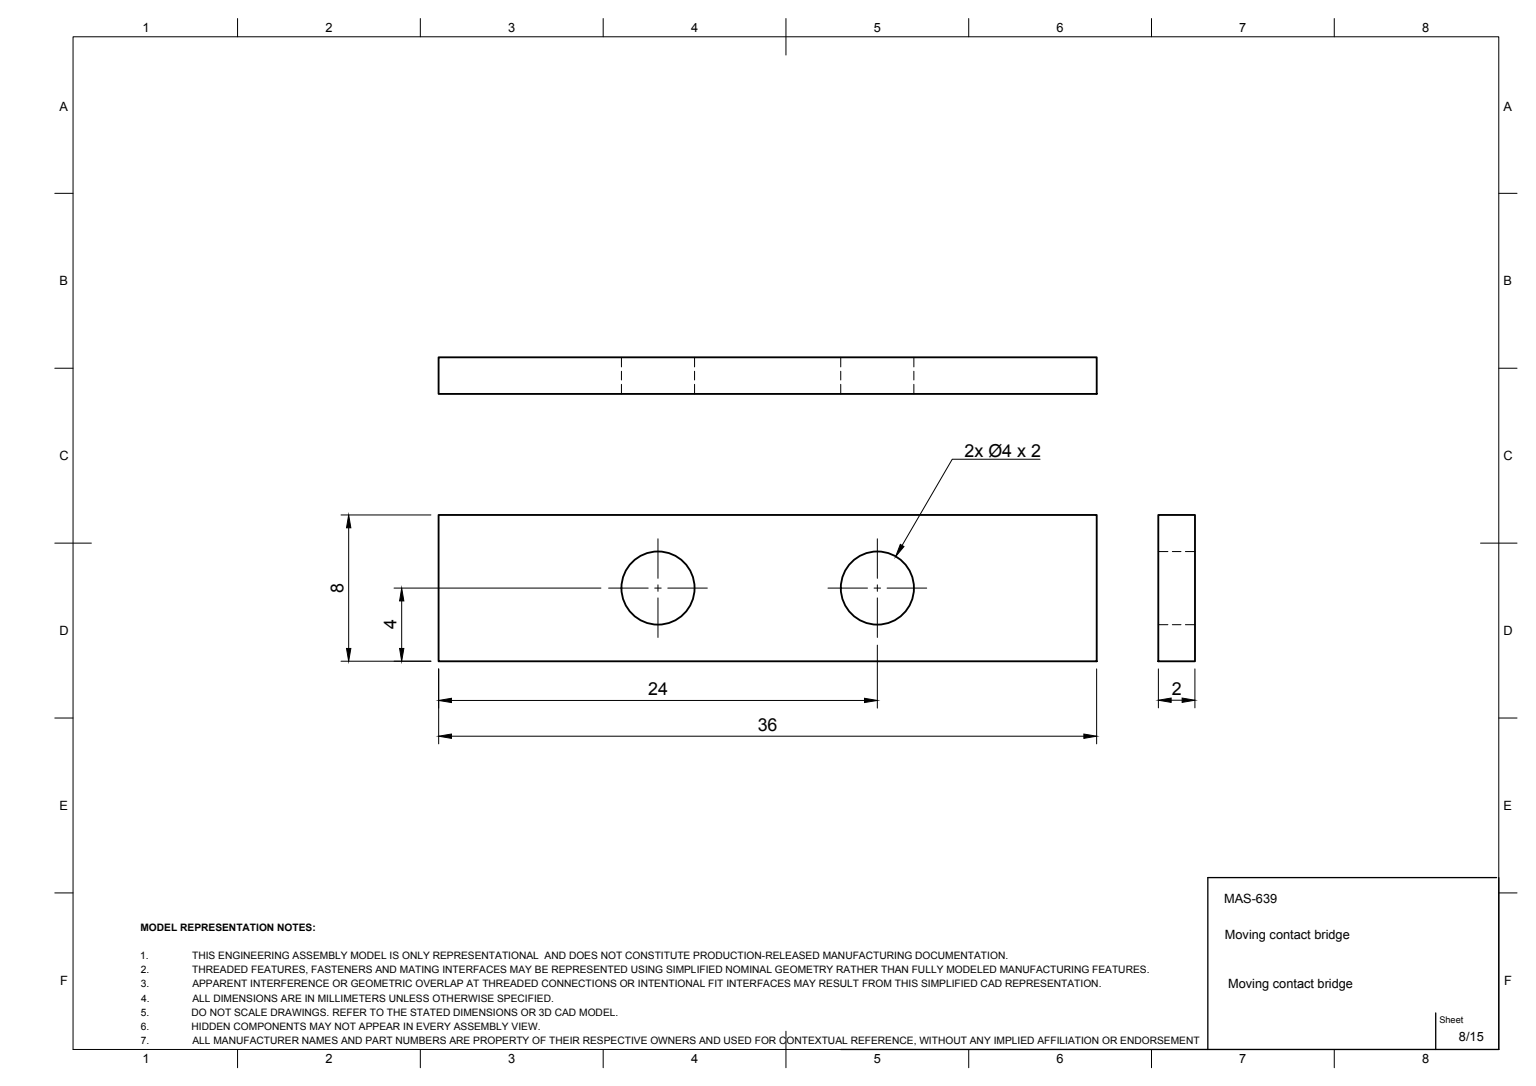
ISO-10303-21;
HEADER;
/* Generated by software containing ST-Developer
 * from STEP Tools, Inc. (www.steptools.com) 
 */

FILE_DESCRIPTION(
/* description */ ('Independent maintained push-to-latch/pull-to-reset mushroom-operator 
CAD. Two opposed spring-loaded ball detents in turned circular seats b
ias both travel stops; direct normally-closed bridge opens6mm when pre
ssed. Rounded palm/pull rim, captured head screw, removable detent clo
sures, native Coil spring families, insulated shared terminals and ord
inary machining features. Manual geometric states and ideal same-mater
ial spring-energy direction only; no electrical/safety certification, 
force/contact dynamics, wear, load or life rating. Requested blue/gray
 visual palette, not safety identification. External wiring/anchors an
d application engineering omitted.'),
/* implementation_level */ '2;1');

FILE_NAME(
/* name */ 'Moving contact bridge.step',
/* time_stamp */ '2026-11-08T17:54:26-08:00',
/* author */ (''),
/* organization */ (''),
/* preprocessor_version */ 'ST-DEVELOPER v20.2',
/* originating_system */ 'Autodesk Translation Framework v15.17.0.0',
/* authorisation */ '');

FILE_SCHEMA (('AUTOMOTIVE_DESIGN { 1 0 10303 214 3 1 1 }'));
ENDSEC;

DATA;
#10=MECHANICAL_DESIGN_GEOMETRIC_PRESENTATION_REPRESENTATION('',(#195),#43980);
#161=SHAPE_REPRESENTATION_RELATIONSHIP('SRR','None',#44061,#178);
#178=ADVANCED_BREP_SHAPE_REPRESENTATION('',(#212),#43968);
#195=STYLED_ITEM('',(#44154),#212);
#212=MANIFOLD_SOLID_BREP('Body1',#11236);
#311=FACE_BOUND('',#1491,.T.);
#312=FACE_BOUND('',#1492,.T.);
#313=FACE_BOUND('',#1494,.T.);
#314=FACE_BOUND('',#1495,.T.);
#405=PLANE('',#11885);
#406=PLANE('',#11886);
#407=PLANE('',#11887);
#408=PLANE('',#11888);
#409=PLANE('',#11889);
#410=PLANE('',#11890);
#809=FACE_OUTER_BOUND('',#1484,.T.);
#810=FACE_OUTER_BOUND('',#1485,.T.);
#811=FACE_OUTER_BOUND('',#1486,.T.);
#812=FACE_OUTER_BOUND('',#1487,.T.);
#813=FACE_OUTER_BOUND('',#1488,.T.);
#814=FACE_OUTER_BOUND('',#1489,.T.);
#815=FACE_OUTER_BOUND('',#1490,.T.);
#816=FACE_OUTER_BOUND('',#1493,.T.);
#1484=EDGE_LOOP('',(#8609,#8610,#8611,#8612));
#1485=EDGE_LOOP('',(#8613,#8614,#8615,#8616));
#1486=EDGE_LOOP('',(#8617,#8618,#8619,#8620));
#1487=EDGE_LOOP('',(#8621,#8622,#8623,#8624));
#1488=EDGE_LOOP('',(#8625,#8626,#8627,#8628));
#1489=EDGE_LOOP('',(#8629,#8630,#8631,#8632));
#1490=EDGE_LOOP('',(#8633,#8634,#8635,#8636));
#1491=EDGE_LOOP('',(#8637));
#1492=EDGE_LOOP('',(#8638));
#1493=EDGE_LOOP('',(#8639,#8640,#8641,#8642));
#1494=EDGE_LOOP('',(#8643));
#1495=EDGE_LOOP('',(#8644));
#1930=CIRCLE('',#11880,0.2);
#1931=CIRCLE('',#11881,0.2);
#1932=CIRCLE('',#11883,0.2);
#1933=CIRCLE('',#11884,0.2);
#3146=LINE('',#29363,#3778);
#3147=LINE('',#29369,#3779);
#3148=LINE('',#29374,#3780);
#3149=LINE('',#29376,#3781);
#3150=LINE('',#29378,#3782);
#3151=LINE('',#29379,#3783);
#3152=LINE('',#29382,#3784);
#3153=LINE('',#29384,#3785);
#3154=LINE('',#29385,#3786);
#3155=LINE('',#29388,#3787);
#3156=LINE('',#29390,#3788);
#3157=LINE('',#29391,#3789);
#3158=LINE('',#29393,#3790);
#3159=LINE('',#29394,#3791);
#3778=VECTOR('',#13473,0.2);
#3779=VECTOR('',#13480,0.2);
#3780=VECTOR('',#13485,1.);
#3781=VECTOR('',#13486,1.);
#3782=VECTOR('',#13487,1.);
#3783=VECTOR('',#13488,1.);
#3784=VECTOR('',#13491,1.);
#3785=VECTOR('',#13492,1.);
#3786=VECTOR('',#13493,1.);
#3787=VECTOR('',#13496,1.);
#3788=VECTOR('',#13497,1.);
#3789=VECTOR('',#13498,1.);
#3790=VECTOR('',#13501,1.);
#3791=VECTOR('',#13502,1.);
#4674=VERTEX_POINT('',#29360);
#4675=VERTEX_POINT('',#29362);
#4676=VERTEX_POINT('',#29366);
#4677=VERTEX_POINT('',#29368);
#4678=VERTEX_POINT('',#29372);
#4679=VERTEX_POINT('',#29373);
#4680=VERTEX_POINT('',#29375);
#4681=VERTEX_POINT('',#29377);
#4682=VERTEX_POINT('',#29381);
#4683=VERTEX_POINT('',#29383);
#4684=VERTEX_POINT('',#29387);
#4685=VERTEX_POINT('',#29389);
#6074=EDGE_CURVE('',#4674,#4674,#1930,.T.);
#6075=EDGE_CURVE('',#4674,#4675,#3146,.T.);
#6076=EDGE_CURVE('',#4675,#4675,#1931,.T.);
#6077=EDGE_CURVE('',#4676,#4676,#1932,.T.);
#6078=EDGE_CURVE('',#4676,#4677,#3147,.T.);
#6079=EDGE_CURVE('',#4677,#4677,#1933,.T.);
#6080=EDGE_CURVE('',#4678,#4679,#3148,.T.);
#6081=EDGE_CURVE('',#4679,#4680,#3149,.T.);
#6082=EDGE_CURVE('',#4681,#4680,#3150,.T.);
#6083=EDGE_CURVE('',#4678,#4681,#3151,.T.);
#6084=EDGE_CURVE('',#4682,#4678,#3152,.T.);
#6085=EDGE_CURVE('',#4683,#4681,#3153,.T.);
#6086=EDGE_CURVE('',#4682,#4683,#3154,.T.);
#6087=EDGE_CURVE('',#4684,#4682,#3155,.T.);
#6088=EDGE_CURVE('',#4685,#4683,#3156,.T.);
#6089=EDGE_CURVE('',#4684,#4685,#3157,.T.);
#6090=EDGE_CURVE('',#4679,#4684,#3158,.T.);
#6091=EDGE_CURVE('',#4680,#4685,#3159,.T.);
#8609=ORIENTED_EDGE('',*,*,#6074,.F.);
#8610=ORIENTED_EDGE('',*,*,#6075,.T.);
#8611=ORIENTED_EDGE('',*,*,#6076,.F.);
#8612=ORIENTED_EDGE('',*,*,#6075,.F.);
#8613=ORIENTED_EDGE('',*,*,#6077,.F.);
#8614=ORIENTED_EDGE('',*,*,#6078,.T.);
#8615=ORIENTED_EDGE('',*,*,#6079,.F.);
#8616=ORIENTED_EDGE('',*,*,#6078,.F.);
#8617=ORIENTED_EDGE('',*,*,#6080,.T.);
#8618=ORIENTED_EDGE('',*,*,#6081,.T.);
#8619=ORIENTED_EDGE('',*,*,#6082,.F.);
#8620=ORIENTED_EDGE('',*,*,#6083,.F.);
#8621=ORIENTED_EDGE('',*,*,#6084,.T.);
#8622=ORIENTED_EDGE('',*,*,#6083,.T.);
#8623=ORIENTED_EDGE('',*,*,#6085,.F.);
#8624=ORIENTED_EDGE('',*,*,#6086,.F.);
#8625=ORIENTED_EDGE('',*,*,#6087,.T.);
#8626=ORIENTED_EDGE('',*,*,#6086,.T.);
#8627=ORIENTED_EDGE('',*,*,#6088,.F.);
#8628=ORIENTED_EDGE('',*,*,#6089,.F.);
#8629=ORIENTED_EDGE('',*,*,#6090,.T.);
#8630=ORIENTED_EDGE('',*,*,#6089,.T.);
#8631=ORIENTED_EDGE('',*,*,#6091,.F.);
#8632=ORIENTED_EDGE('',*,*,#6081,.F.);
#8633=ORIENTED_EDGE('',*,*,#6091,.T.);
#8634=ORIENTED_EDGE('',*,*,#6088,.T.);
#8635=ORIENTED_EDGE('',*,*,#6085,.T.);
#8636=ORIENTED_EDGE('',*,*,#6082,.T.);
#8637=ORIENTED_EDGE('',*,*,#6074,.T.);
#8638=ORIENTED_EDGE('',*,*,#6077,.T.);
#8639=ORIENTED_EDGE('',*,*,#6090,.F.);
#8640=ORIENTED_EDGE('',*,*,#6080,.F.);
#8641=ORIENTED_EDGE('',*,*,#6084,.F.);
#8642=ORIENTED_EDGE('',*,*,#6087,.F.);
#8643=ORIENTED_EDGE('',*,*,#6076,.T.);
#8644=ORIENTED_EDGE('',*,*,#6079,.T.);
#10412=CYLINDRICAL_SURFACE('',#11879,0.2);
#10413=CYLINDRICAL_SURFACE('',#11882,0.2);
#10934=ADVANCED_FACE('',(#809),#10412,.F.);
#10935=ADVANCED_FACE('',(#810),#10413,.F.);
#10936=ADVANCED_FACE('',(#811),#405,.T.);
#10937=ADVANCED_FACE('',(#812),#406,.T.);
#10938=ADVANCED_FACE('',(#813),#407,.T.);
#10939=ADVANCED_FACE('',(#814),#408,.T.);
#10940=ADVANCED_FACE('',(#815,#311,#312),#409,.T.);
#10941=ADVANCED_FACE('',(#816,#313,#314),#410,.F.);
#11236=CLOSED_SHELL('',(#10934,#10935,#10936,#10937,#10938,#10939,#10940,
#10941));
#11878=AXIS2_PLACEMENT_3D('',#29358,#13467,#13468);
#11879=AXIS2_PLACEMENT_3D('',#29359,#13469,#13470);
#11880=AXIS2_PLACEMENT_3D('',#29361,#13471,#13472);
#11881=AXIS2_PLACEMENT_3D('',#29364,#13474,#13475);
#11882=AXIS2_PLACEMENT_3D('',#29365,#13476,#13477);
#11883=AXIS2_PLACEMENT_3D('',#29367,#13478,#13479);
#11884=AXIS2_PLACEMENT_3D('',#29370,#13481,#13482);
#11885=AXIS2_PLACEMENT_3D('',#29371,#13483,#13484);
#11886=AXIS2_PLACEMENT_3D('',#29380,#13489,#13490);
#11887=AXIS2_PLACEMENT_3D('',#29386,#13494,#13495);
#11888=AXIS2_PLACEMENT_3D('',#29392,#13499,#13500);
#11889=AXIS2_PLACEMENT_3D('',#29395,#13503,#13504);
#11890=AXIS2_PLACEMENT_3D('',#29396,#13505,#13506);
#13467=DIRECTION('axis',(0.,0.,1.));
#13468=DIRECTION('refdir',(1.,0.,0.));
#13469=DIRECTION('center_axis',(0.,0.,-1.));
#13470=DIRECTION('ref_axis',(1.,0.,0.));
#13471=DIRECTION('center_axis',(0.,0.,-1.));
#13472=DIRECTION('ref_axis',(1.,0.,0.));
#13473=DIRECTION('',(0.,0.,-1.));
#13474=DIRECTION('center_axis',(0.,0.,1.));
#13475=DIRECTION('ref_axis',(1.,0.,0.));
#13476=DIRECTION('center_axis',(0.,0.,-1.));
#13477=DIRECTION('ref_axis',(1.,0.,0.));
#13478=DIRECTION('center_axis',(0.,0.,-1.));
#13479=DIRECTION('ref_axis',(1.,0.,0.));
#13480=DIRECTION('',(0.,0.,-1.));
#13481=DIRECTION('center_axis',(0.,0.,1.));
#13482=DIRECTION('ref_axis',(1.,0.,0.));
#13483=DIRECTION('center_axis',(0.,1.,0.));
#13484=DIRECTION('ref_axis',(-1.,0.,0.));
#13485=DIRECTION('',(-1.,0.,0.));
#13486=DIRECTION('',(0.,0.,1.));
#13487=DIRECTION('',(-1.,0.,0.));
#13488=DIRECTION('',(0.,0.,1.));
#13489=DIRECTION('center_axis',(1.,0.,0.));
#13490=DIRECTION('ref_axis',(0.,1.,0.));
#13491=DIRECTION('',(0.,1.,0.));
#13492=DIRECTION('',(0.,1.,0.));
#13493=DIRECTION('',(0.,0.,1.));
#13494=DIRECTION('center_axis',(0.,-1.,0.));
#13495=DIRECTION('ref_axis',(1.,0.,0.));
#13496=DIRECTION('',(1.,0.,0.));
#13497=DIRECTION('',(1.,0.,0.));
#13498=DIRECTION('',(0.,0.,1.));
#13499=DIRECTION('center_axis',(-1.,0.,0.));
#13500=DIRECTION('ref_axis',(0.,-1.,0.));
#13501=DIRECTION('',(0.,-1.,0.));
#13502=DIRECTION('',(0.,-1.,0.));
#13503=DIRECTION('center_axis',(0.,0.,1.));
#13504=DIRECTION('ref_axis',(1.,0.,0.));
#13505=DIRECTION('center_axis',(0.,0.,1.));
#13506=DIRECTION('ref_axis',(1.,0.,0.));
#29358=CARTESIAN_POINT('',(0.,0.,0.));
#29359=CARTESIAN_POINT('Origin',(-0.6,1.,2.5));
#29360=CARTESIAN_POINT('',(-0.8,1.,2.6));
#29361=CARTESIAN_POINT('Origin',(-0.6,1.,2.6));
#29362=CARTESIAN_POINT('',(-0.8,1.,2.4));
#29363=CARTESIAN_POINT('',(-0.8,1.,2.5));
#29364=CARTESIAN_POINT('Origin',(-0.6,1.,2.4));
#29365=CARTESIAN_POINT('Origin',(0.6,1.,2.5));
#29366=CARTESIAN_POINT('',(0.4,1.,2.6));
#29367=CARTESIAN_POINT('Origin',(0.6,1.,2.6));
#29368=CARTESIAN_POINT('',(0.4,1.,2.4));
#29369=CARTESIAN_POINT('',(0.4,1.,2.5));
#29370=CARTESIAN_POINT('Origin',(0.6,1.,2.4));
#29371=CARTESIAN_POINT('Origin',(1.8,1.4,2.4));
#29372=CARTESIAN_POINT('',(1.8,1.4,2.4));
#29373=CARTESIAN_POINT('',(-1.8,1.4,2.4));
#29374=CARTESIAN_POINT('',(1.8,1.4,2.4));
#29375=CARTESIAN_POINT('',(-1.8,1.4,2.6));
#29376=CARTESIAN_POINT('',(-1.8,1.4,2.4));
#29377=CARTESIAN_POINT('',(1.8,1.4,2.6));
#29378=CARTESIAN_POINT('',(1.8,1.4,2.6));
#29379=CARTESIAN_POINT('',(1.8,1.4,2.4));
#29380=CARTESIAN_POINT('Origin',(1.8,0.6,2.4));
#29381=CARTESIAN_POINT('',(1.8,0.6,2.4));
#29382=CARTESIAN_POINT('',(1.8,0.6,2.4));
#29383=CARTESIAN_POINT('',(1.8,0.6,2.6));
#29384=CARTESIAN_POINT('',(1.8,0.6,2.6));
#29385=CARTESIAN_POINT('',(1.8,0.6,2.4));
#29386=CARTESIAN_POINT('Origin',(-1.8,0.6,2.4));
#29387=CARTESIAN_POINT('',(-1.8,0.6,2.4));
#29388=CARTESIAN_POINT('',(-1.8,0.6,2.4));
#29389=CARTESIAN_POINT('',(-1.8,0.6,2.6));
#29390=CARTESIAN_POINT('',(-1.8,0.6,2.6));
#29391=CARTESIAN_POINT('',(-1.8,0.6,2.4));
#29392=CARTESIAN_POINT('Origin',(-1.8,1.4,2.4));
#29393=CARTESIAN_POINT('',(-1.8,1.4,2.4));
#29394=CARTESIAN_POINT('',(-1.8,1.4,2.6));
#29395=CARTESIAN_POINT('Origin',(0.,1.,2.6));
#29396=CARTESIAN_POINT('Origin',(0.,1.,2.4));
#43949=UNCERTAINTY_MEASURE_WITH_UNIT(LENGTH_MEASURE(0.001),#43981,
'DISTANCE_ACCURACY_VALUE',
'Maximum model space distance between geometric entities at asserted c
onnectivities');
#43961=UNCERTAINTY_MEASURE_WITH_UNIT(LENGTH_MEASURE(0.001),#43981,
'DISTANCE_ACCURACY_VALUE',
'Maximum model space distance between geometric entities at asserted c
onnectivities');
#43968=(
GEOMETRIC_REPRESENTATION_CONTEXT(3)
GLOBAL_UNCERTAINTY_ASSIGNED_CONTEXT((#43949))
GLOBAL_UNIT_ASSIGNED_CONTEXT((#43981,#43983,#43984))
REPRESENTATION_CONTEXT('','3D')
);
#43980=(
GEOMETRIC_REPRESENTATION_CONTEXT(3)
GLOBAL_UNCERTAINTY_ASSIGNED_CONTEXT((#43961))
GLOBAL_UNIT_ASSIGNED_CONTEXT((#43981,#43983,#43984))
REPRESENTATION_CONTEXT('','3D')
);
#43981=(
LENGTH_UNIT()
NAMED_UNIT(*)
SI_UNIT(.CENTI.,.METRE.)
);
#43983=(
NAMED_UNIT(*)
PLANE_ANGLE_UNIT()
SI_UNIT($,.RADIAN.)
);
#43984=(
NAMED_UNIT(*)
SI_UNIT($,.STERADIAN.)
SOLID_ANGLE_UNIT()
);
#43991=SHAPE_DEFINITION_REPRESENTATION(#44009,#44061);
#44009=PRODUCT_DEFINITION_SHAPE('',$,#44080);
#44061=SHAPE_REPRESENTATION('',(#11878),#43968);
#44073=PRODUCT_DEFINITION_CONTEXT('part definition',#44129,'design');
#44080=PRODUCT_DEFINITION('Moving contact bridge',
'Moving contact bridge',#44098,#44073);
#44098=PRODUCT_DEFINITION_FORMATION('',$,#44137);
#44129=APPLICATION_CONTEXT(
'Core Data for Automotive Mechanical Design Process');
#44130=PRODUCT_CONTEXT('part definition',#44129,'mechanical');
#44137=PRODUCT('Moving contact bridge','Moving contact bridge',$,(#44130));
#44154=PRESENTATION_STYLE_ASSIGNMENT((#44166));
#44166=SURFACE_STYLE_USAGE(.BOTH.,#44178);
#44178=SURFACE_SIDE_STYLE('',(#44190));
#44190=SURFACE_STYLE_FILL_AREA(#44202);
#44202=FILL_AREA_STYLE('Contact gray',(#44214));
#44214=FILL_AREA_STYLE_COLOUR('Contact gray',#44226);
#44226=COLOUR_RGB('Contact gray',0.725490196078431,0.752941176470588,0.792156862745098);
ENDSEC;
END-ISO-10303-21;
